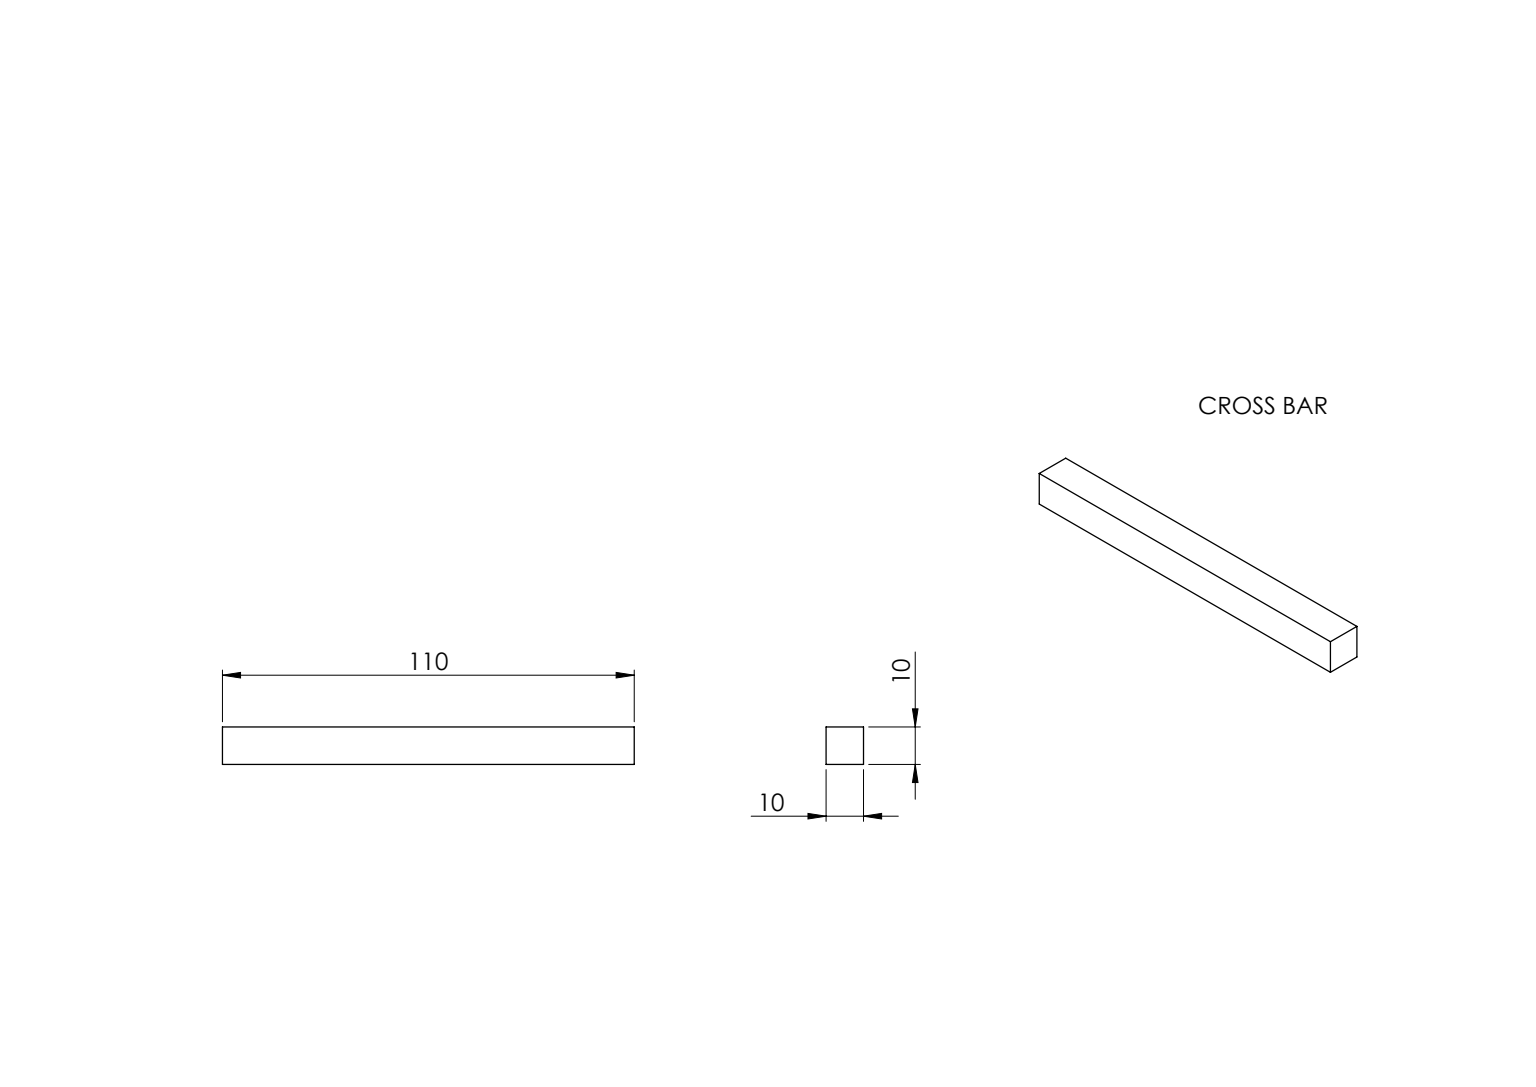
ISO-10303-21;
HEADER;
FILE_DESCRIPTION (('STEP AP214'),
    '1' );
FILE_NAME ('cross bar.step',
    '2026-10-24T04:45:50',
    ( '' ),
    ( '' ),
    'SwSTEP 2.0',
    'SolidWorks 2026',
    '' );
FILE_SCHEMA (( 'AUTOMOTIVE_DESIGN' ));
ENDSEC;

DATA;
#1=ADVANCED_BREP_SHAPE_REPRESENTATION ( '', ( #1992, #3111 ), #2618 ) ;
#17=DIRECTION ( 'NONE',  ( 0.000000000000000000, 0.000000000000000000, -1.000000000000000000 ) ) ;
#38=VERTEX_POINT ( 'NONE', #2461 ) ;
#78=VERTEX_POINT ( 'NONE', #1445 ) ;
#107=SHAPE_REPRESENTATION ( 'cross bar', ( #3111 ), #2618 ) ;
#112=APPLICATION_CONTEXT ( 'automotive_design' ) ;
#116=DIRECTION ( 'NONE',  ( 4.857225732735056709E-15, 0.000000000000000000, 1.000000000000000000 ) ) ;
#140=UNCERTAINTY_MEASURE_WITH_UNIT (LENGTH_MEASURE( 1.000000000000000082E-05 ), #3331, 'distance_accuracy_value', 'NONE');
#162=EDGE_LOOP ( 'NONE', ( #2034, #1285, #2151, #1503 ) ) ;
#193=DIRECTION ( 'NONE',  ( -4.857225732735056709E-15, 0.000000000000000000, -1.000000000000000000 ) ) ;
#228=( NAMED_UNIT ( * ) SI_UNIT ( $, .STERADIAN. ) SOLID_ANGLE_UNIT ( ) );
#236=ADVANCED_FACE ( 'NONE', ( #2285 ), #2096, .F. ) ;
#243=EDGE_LOOP ( 'NONE', ( #2805, #1759, #1997, #2614 ) ) ;
#271=VECTOR ( 'NONE', #3335, 1000.000000000000000 ) ;
#287=APPLICATION_CONTEXT ( 'automotive_design' ) ;
#289=FACE_OUTER_BOUND ( 'NONE', #2539, .T. ) ;
#351=DIRECTION ( 'NONE',  ( 0.000000000000000000, 0.000000000000000000, -1.000000000000000000 ) ) ;
#365=MECHANICAL_DESIGN_GEOMETRIC_PRESENTATION_REPRESENTATION('',(#2220),#1676);
#384=STYLED_ITEM ( 'NONE', ( #3081 ), #1 ) ;
#398=ORIENTED_EDGE ( 'NONE', *, *, #2812, .T. ) ;
#410=DIRECTION ( 'NONE',  ( -1.000000000000000000, -0.000000000000000000, 2.365532012695647326E-17 ) ) ;
#417=CARTESIAN_POINT ( 'NONE',  ( 55.00000000000000000, 130.0000000000000000, -5.000000000000000000 ) ) ;
#441=CARTESIAN_POINT ( 'NONE',  ( 55.00000000000004974, 130.0000000000000000, 5.000000000000004441 ) ) ;
#452=ADVANCED_FACE ( 'NONE', ( #1953 ), #2723, .F. ) ;
#457=CARTESIAN_POINT ( 'NONE',  ( -54.99999999999995026, 120.0000000000000142, 5.000000000000004441 ) ) ;
#485=VECTOR ( 'NONE', #1029, 1000.000000000000000 ) ;
#521=CARTESIAN_POINT ( 'NONE',  ( 0.000000000000000000, 120.0000000000000142, 0.000000000000000000 ) ) ;
#541=PLANE ( 'NONE',  #2013 ) ;
#559=CARTESIAN_POINT ( 'NONE',  ( 0.000000000000000000, 130.0000000000000000, 0.000000000000000000 ) ) ;
#581=UNCERTAINTY_MEASURE_WITH_UNIT (LENGTH_MEASURE( 1.000000000000000082E-05 ), #795, 'distance_accuracy_value', 'NONE');
#653=COLOUR_RGB ( '',0.8941176470588234615, 0.8941176470588234615, 0.8941176470588234615 ) ;
#669=PRODUCT_CONTEXT ( 'NONE', #112, 'mechanical' ) ;
#680=DIRECTION ( 'NONE',  ( -1.000000000000000000, -0.000000000000000000, 2.365532012695647326E-17 ) ) ;
#691=EDGE_CURVE ( 'NONE', #902, #38, #3333, .T. ) ;
#720=CARTESIAN_POINT ( 'NONE',  ( 55.00000000000004974, 120.0000000000000142, 5.000000000000004441 ) ) ;
#741=EDGE_CURVE ( 'NONE', #2732, #2342, #2193, .T. ) ;
#762=SURFACE_STYLE_USAGE ( .BOTH. , #1583 ) ;
#784=DIRECTION ( 'NONE',  ( -0.000000000000000000, -0.000000000000000000, 1.000000000000000000 ) ) ;
#786=DIRECTION ( 'NONE',  ( -4.857225732735056709E-15, 0.000000000000000000, -1.000000000000000000 ) ) ;
#795=( LENGTH_UNIT ( ) NAMED_UNIT ( * ) SI_UNIT ( .MILLI., .METRE. ) );
#816=VECTOR ( 'NONE', #3084, 1000.000000000000000 ) ;
#902=VERTEX_POINT ( 'NONE', #720 ) ;
#907=EDGE_CURVE ( 'NONE', #38, #2342, #2800, .T. ) ;
#912=VECTOR ( 'NONE', #2702, 1000.000000000000000 ) ;
#920=DIRECTION ( 'NONE',  ( 0.000000000000000000, 0.000000000000000000, -1.000000000000000000 ) ) ;
#928=AXIS2_PLACEMENT_3D ( 'NONE', #2519, #1495, #920 ) ;
#935=PLANE ( 'NONE',  #2763 ) ;
#942=DIRECTION ( 'NONE',  ( -0.000000000000000000, -0.000000000000000000, 1.000000000000000000 ) ) ;
#972=LINE ( 'NONE', #1433, #1410 ) ;
#1001=ORIENTED_EDGE ( 'NONE', *, *, #2906, .T. ) ;
#1029=DIRECTION ( 'NONE',  ( 1.000000000000000000, 0.000000000000000000, 0.000000000000000000 ) ) ;
#1039=VECTOR ( 'NONE', #942, 1000.000000000000000 ) ;
#1056=( LENGTH_UNIT ( ) NAMED_UNIT ( * ) SI_UNIT ( .MILLI., .METRE. ) );
#1060=DIRECTION ( 'NONE',  ( 0.000000000000000000, -1.000000000000000000, 0.000000000000000000 ) ) ;
#1118=EDGE_CURVE ( 'NONE', #2239, #78, #1287, .T. ) ;
#1124=ORIENTED_EDGE ( 'NONE', *, *, #1387, .T. ) ;
#1131=FACE_OUTER_BOUND ( 'NONE', #2670, .T. ) ;
#1142=VECTOR ( 'NONE', #1386, 1000.000000000000000 ) ;
#1155=MECHANICAL_DESIGN_GEOMETRIC_PRESENTATION_REPRESENTATION('',(#384),#2399);
#1169=ORIENTED_EDGE ( 'NONE', *, *, #1118, .F. ) ;
#1195=VECTOR ( 'NONE', #680, 1000.000000000000000 ) ;
#1207=PRODUCT_DEFINITION_CONTEXT ( 'detailed design', #287, 'design' ) ;
#1225=CARTESIAN_POINT ( 'NONE',  ( -54.99999999999995026, 130.0000000000000000, 5.000000000000004441 ) ) ;
#1237=ORIENTED_EDGE ( 'NONE', *, *, #741, .T. ) ;
#1239=SURFACE_STYLE_FILL_AREA ( #3099 ) ;
#1264=SHAPE_REPRESENTATION_RELATIONSHIP ( 'NONE' , 'NONE' ,  #107, #1 ) ;
#1285=ORIENTED_EDGE ( 'NONE', *, *, #1701, .F. ) ;
#1287=LINE ( 'NONE', #3371, #485 ) ;
#1295=DIRECTION ( 'NONE',  ( 2.365532012695647018E-17, -0.000000000000000000, 1.000000000000000000 ) ) ;
#1309=FILL_AREA_STYLE_COLOUR ( '', #653 ) ;
#1372=CARTESIAN_POINT ( 'NONE',  ( -54.99999999999995026, 130.0000000000000000, -4.999999999999997335 ) ) ;
#1386=DIRECTION ( 'NONE',  ( -0.000000000000000000, -1.000000000000000000, -0.000000000000000000 ) ) ;
#1387=EDGE_CURVE ( 'NONE', #2306, #2732, #972, .T. ) ;
#1410=VECTOR ( 'NONE', #410, 1000.000000000000000 ) ;
#1414=AXIS2_PLACEMENT_3D ( 'NONE', #559, #2370, #351 ) ;
#1426=SHAPE_DEFINITION_REPRESENTATION ( #1977, #107 ) ;
#1427=ORIENTED_EDGE ( 'NONE', *, *, #907, .F. ) ;
#1433=CARTESIAN_POINT ( 'NONE',  ( -54.99999999999995026, 130.0000000000000000, -4.999999999999997335 ) ) ;
#1445=CARTESIAN_POINT ( 'NONE',  ( 55.00000000000004974, 130.0000000000000000, 5.000000000000004441 ) ) ;
#1448=EDGE_CURVE ( 'NONE', #2342, #2464, #1467, .T. ) ;
#1467=LINE ( 'NONE', #3337, #2121 ) ;
#1472=UNCERTAINTY_MEASURE_WITH_UNIT (LENGTH_MEASURE( 1.000000000000000082E-05 ), #1056, 'distance_accuracy_value', 'NONE');
#1495=DIRECTION ( 'NONE',  ( 1.000000000000000000, -0.000000000000000000, 0.000000000000000000 ) ) ;
#1501=CARTESIAN_POINT ( 'NONE',  ( -54.99999999999995026, 120.0000000000000142, -4.999999999999997335 ) ) ;
#1503=ORIENTED_EDGE ( 'NONE', *, *, #3252, .T. ) ;
#1505=ORIENTED_EDGE ( 'NONE', *, *, #1448, .T. ) ;
#1507=AXIS2_PLACEMENT_3D ( 'NONE', #3336, #1295, #2333 ) ;
#1583=SURFACE_SIDE_STYLE ('',( #1239 ) ) ;
#1587=PRODUCT_DEFINITION_FORMATION_WITH_SPECIFIED_SOURCE ( 'ANY', '', #1790, .NOT_KNOWN. ) ;
#1648=ORIENTED_EDGE ( 'NONE', *, *, #1448, .F. ) ;
#1658=CARTESIAN_POINT ( 'NONE',  ( -54.99999999999995026, 130.0000000000000000, -4.999999999999997335 ) ) ;
#1666=CARTESIAN_POINT ( 'NONE',  ( 55.00000000000000000, 130.0000000000000000, -5.000000000000000000 ) ) ;
#1676=( GEOMETRIC_REPRESENTATION_CONTEXT ( 3 ) GLOBAL_UNCERTAINTY_ASSIGNED_CONTEXT ( ( #581 ) ) GLOBAL_UNIT_ASSIGNED_CONTEXT ( ( #795, #2859, #3124 ) ) REPRESENTATION_CONTEXT ( 'NONE', 'WORKASPACE' ) );
#1690=PLANE ( 'NONE',  #928 ) ;
#1701=EDGE_CURVE ( 'NONE', #2306, #38, #1887, .T. ) ;
#1715=DIRECTION ( 'NONE',  ( 0.000000000000000000, 0.000000000000000000, -1.000000000000000000 ) ) ;
#1721=EDGE_CURVE ( 'NONE', #2239, #2464, #2688, .T. ) ;
#1754=ADVANCED_FACE ( 'NONE', ( #1131 ), #2164, .F. ) ;
#1759=ORIENTED_EDGE ( 'NONE', *, *, #741, .F. ) ;
#1769=LINE ( 'NONE', #2807, #816 ) ;
#1775=ORIENTED_EDGE ( 'NONE', *, *, #3153, .F. ) ;
#1790=PRODUCT ( 'cross bar', 'cross bar', '', ( #669 ) ) ;
#1795=ORIENTED_EDGE ( 'NONE', *, *, #2812, .F. ) ;
#1839=LINE ( 'NONE', #3368, #2994 ) ;
#1871=CARTESIAN_POINT ( 'NONE',  ( 0.000000000000000000, 0.000000000000000000, 0.000000000000000000 ) ) ;
#1887=LINE ( 'NONE', #1666, #912 ) ;
#1924=CARTESIAN_POINT ( 'NONE',  ( -54.99999999999995026, 130.0000000000000000, 5.000000000000004441 ) ) ;
#1934=EDGE_LOOP ( 'NONE', ( #1505, #2516, #1795, #1237 ) ) ;
#1953=FACE_OUTER_BOUND ( 'NONE', #162, .T. ) ;
#1969=CARTESIAN_POINT ( 'NONE',  ( -54.99999999999995026, 130.0000000000000000, 5.000000000000004441 ) ) ;
#1977=PRODUCT_DEFINITION_SHAPE ( 'NONE', 'NONE',  #3197 ) ;
#1992=MANIFOLD_SOLID_BREP ( 'Boss-Extrude1', #2753 ) ;
#1997=ORIENTED_EDGE ( 'NONE', *, *, #1387, .F. ) ;
#2013=AXIS2_PLACEMENT_3D ( 'NONE', #521, #1060, #17 ) ;
#2034=ORIENTED_EDGE ( 'NONE', *, *, #691, .T. ) ;
#2042=( NAMED_UNIT ( * ) PLANE_ANGLE_UNIT ( ) SI_UNIT ( $, .RADIAN. ) );
#2096=PLANE ( 'NONE',  #1507 ) ;
#2121=VECTOR ( 'NONE', #784, 1000.000000000000000 ) ;
#2126=VECTOR ( 'NONE', #3194, 1000.000000000000000 ) ;
#2151=ORIENTED_EDGE ( 'NONE', *, *, #2906, .F. ) ;
#2164=PLANE ( 'NONE',  #1414 ) ;
#2184=DIRECTION ( 'NONE',  ( -1.000000000000000000, 0.000000000000000000, 4.857225732735056709E-15 ) ) ;
#2193=LINE ( 'NONE', #1372, #1142 ) ;
#2220=STYLED_ITEM('',(#3408),#1992);
#2224=VECTOR ( 'NONE', #193, 1000.000000000000000 ) ;
#2239=VERTEX_POINT ( 'NONE', #1225 ) ;
#2241=DIRECTION ( 'NONE',  ( -1.000000000000000000, 0.000000000000000000, -0.000000000000000000 ) ) ;
#2285=FACE_OUTER_BOUND ( 'NONE', #243, .T. ) ;
#2306=VERTEX_POINT ( 'NONE', #417 ) ;
#2333=DIRECTION ( 'NONE',  ( 1.000000000000000000, 0.000000000000000000, -2.365532012695647018E-17 ) ) ;
#2342=VERTEX_POINT ( 'NONE', #3291 ) ;
#2370=DIRECTION ( 'NONE',  ( 0.000000000000000000, -1.000000000000000000, 0.000000000000000000 ) ) ;
#2371=ADVANCED_FACE ( 'NONE', ( #3277 ), #935, .F. ) ;
#2390=ORIENTED_EDGE ( 'NONE', *, *, #1118, .T. ) ;
#2399=( GEOMETRIC_REPRESENTATION_CONTEXT ( 3 ) GLOBAL_UNCERTAINTY_ASSIGNED_CONTEXT ( ( #140 ) ) GLOBAL_UNIT_ASSIGNED_CONTEXT ( ( #3331, #2042, #3136 ) ) REPRESENTATION_CONTEXT ( 'NONE', 'WORKASPACE' ) );
#2461=CARTESIAN_POINT ( 'NONE',  ( 55.00000000000000000, 120.0000000000000142, -5.000000000000000000 ) ) ;
#2464=VERTEX_POINT ( 'NONE', #2527 ) ;
#2473=LINE ( 'NONE', #457, #271 ) ;
#2508=LINE ( 'NONE', #3059, #1039 ) ;
#2516=ORIENTED_EDGE ( 'NONE', *, *, #1721, .F. ) ;
#2519=CARTESIAN_POINT ( 'NONE',  ( -54.99999999999995026, 130.0000000000000000, 5.000000000000004441 ) ) ;
#2527=CARTESIAN_POINT ( 'NONE',  ( -54.99999999999995026, 120.0000000000000142, 5.000000000000004441 ) ) ;
#2539=EDGE_LOOP ( 'NONE', ( #3060, #1775, #1648, #1427 ) ) ;
#2614=ORIENTED_EDGE ( 'NONE', *, *, #1701, .T. ) ;
#2618=( GEOMETRIC_REPRESENTATION_CONTEXT ( 3 ) GLOBAL_UNCERTAINTY_ASSIGNED_CONTEXT ( ( #1472 ) ) GLOBAL_UNIT_ASSIGNED_CONTEXT ( ( #1056, #3345, #228 ) ) REPRESENTATION_CONTEXT ( 'NONE', 'WORKASPACE' ) );
#2639=DIRECTION ( 'NONE',  ( 1.000000000000000000, 0.000000000000000000, 0.000000000000000000 ) ) ;
#2670=EDGE_LOOP ( 'NONE', ( #1001, #1124, #398, #2390 ) ) ;
#2688=LINE ( 'NONE', #1924, #2126 ) ;
#2702=DIRECTION ( 'NONE',  ( -0.000000000000000000, -1.000000000000000000, -0.000000000000000000 ) ) ;
#2723=PLANE ( 'NONE',  #2986 ) ;
#2732=VERTEX_POINT ( 'NONE', #1658 ) ;
#2753=CLOSED_SHELL ( 'NONE', ( #452, #236, #3173, #2371, #1754, #3244 ) ) ;
#2763=AXIS2_PLACEMENT_3D ( 'NONE', #1969, #1715, #2241 ) ;
#2789=CARTESIAN_POINT ( 'NONE',  ( 55.00000000000004974, 120.0000000000000142, 5.000000000000004441 ) ) ;
#2800=LINE ( 'NONE', #1501, #1195 ) ;
#2805=ORIENTED_EDGE ( 'NONE', *, *, #907, .T. ) ;
#2807=CARTESIAN_POINT ( 'NONE',  ( 55.00000000000004974, 130.0000000000000000, 5.000000000000004441 ) ) ;
#2812=EDGE_CURVE ( 'NONE', #2732, #2239, #2508, .T. ) ;
#2859=( NAMED_UNIT ( * ) PLANE_ANGLE_UNIT ( ) SI_UNIT ( $, .RADIAN. ) );
#2866=EDGE_LOOP ( 'NONE', ( #2916, #3354, #1169, #2917 ) ) ;
#2906=EDGE_CURVE ( 'NONE', #78, #2306, #1839, .T. ) ;
#2916=ORIENTED_EDGE ( 'NONE', *, *, #3153, .T. ) ;
#2917=ORIENTED_EDGE ( 'NONE', *, *, #1721, .T. ) ;
#2986=AXIS2_PLACEMENT_3D ( 'NONE', #441, #2184, #116 ) ;
#2994=VECTOR ( 'NONE', #786, 1000.000000000000000 ) ;
#3059=CARTESIAN_POINT ( 'NONE',  ( -54.99999999999995026, 130.0000000000000000, 5.000000000000004441 ) ) ;
#3060=ORIENTED_EDGE ( 'NONE', *, *, #691, .F. ) ;
#3081=PRESENTATION_STYLE_ASSIGNMENT (( #762 ) ) ;
#3084=DIRECTION ( 'NONE',  ( -0.000000000000000000, -1.000000000000000000, -0.000000000000000000 ) ) ;
#3099=FILL_AREA_STYLE ('',( #1309 ) ) ;
#3111=AXIS2_PLACEMENT_3D ( 'NONE', #1871, #3207, #2639 ) ;
#3124=( NAMED_UNIT ( * ) SI_UNIT ( $, .STERADIAN. ) SOLID_ANGLE_UNIT ( ) );
#3136=( NAMED_UNIT ( * ) SI_UNIT ( $, .STERADIAN. ) SOLID_ANGLE_UNIT ( ) );
#3153=EDGE_CURVE ( 'NONE', #2464, #902, #2473, .T. ) ;
#3173=ADVANCED_FACE ( 'NONE', ( #3263 ), #1690, .F. ) ;
#3194=DIRECTION ( 'NONE',  ( -0.000000000000000000, -1.000000000000000000, -0.000000000000000000 ) ) ;
#3197=PRODUCT_DEFINITION ( 'UNKNOWN', '', #1587, #1207 ) ;
#3207=DIRECTION ( 'NONE',  ( 0.000000000000000000, 0.000000000000000000, 1.000000000000000000 ) ) ;
#3244=ADVANCED_FACE ( 'NONE', ( #289 ), #541, .T. ) ;
#3252=EDGE_CURVE ( 'NONE', #78, #902, #1769, .T. ) ;
#3263=FACE_OUTER_BOUND ( 'NONE', #1934, .T. ) ;
#3277=FACE_OUTER_BOUND ( 'NONE', #2866, .T. ) ;
#3291=CARTESIAN_POINT ( 'NONE',  ( -54.99999999999995026, 120.0000000000000142, -4.999999999999997335 ) ) ;
#3331=( LENGTH_UNIT ( ) NAMED_UNIT ( * ) SI_UNIT ( .MILLI., .METRE. ) );
#3333=LINE ( 'NONE', #2789, #2224 ) ;
#3335=DIRECTION ( 'NONE',  ( 1.000000000000000000, 0.000000000000000000, 0.000000000000000000 ) ) ;
#3336=CARTESIAN_POINT ( 'NONE',  ( -54.99999999999995026, 130.0000000000000000, -4.999999999999997335 ) ) ;
#3337=CARTESIAN_POINT ( 'NONE',  ( -54.99999999999995026, 120.0000000000000142, 5.000000000000004441 ) ) ;
#3345=( NAMED_UNIT ( * ) PLANE_ANGLE_UNIT ( ) SI_UNIT ( $, .RADIAN. ) );
#3354=ORIENTED_EDGE ( 'NONE', *, *, #3252, .F. ) ;
#3368=CARTESIAN_POINT ( 'NONE',  ( 55.00000000000004974, 130.0000000000000000, 5.000000000000004441 ) ) ;
#3371=CARTESIAN_POINT ( 'NONE',  ( -54.99999999999995026, 130.0000000000000000, 5.000000000000004441 ) ) ;
#3402=COLOUR_RGB('Sky Blue',0.24,0.69,0.87);
#3403=FILL_AREA_STYLE_COLOUR('',#3402);
#3404=FILL_AREA_STYLE('',(#3403));
#3405=SURFACE_STYLE_FILL_AREA(#3404);
#3406=SURFACE_SIDE_STYLE('',(#3405));
#3407=SURFACE_STYLE_USAGE(.BOTH.,#3406);
#3408=PRESENTATION_STYLE_ASSIGNMENT((#3407));
ENDSEC;
END-ISO-10303-21;
